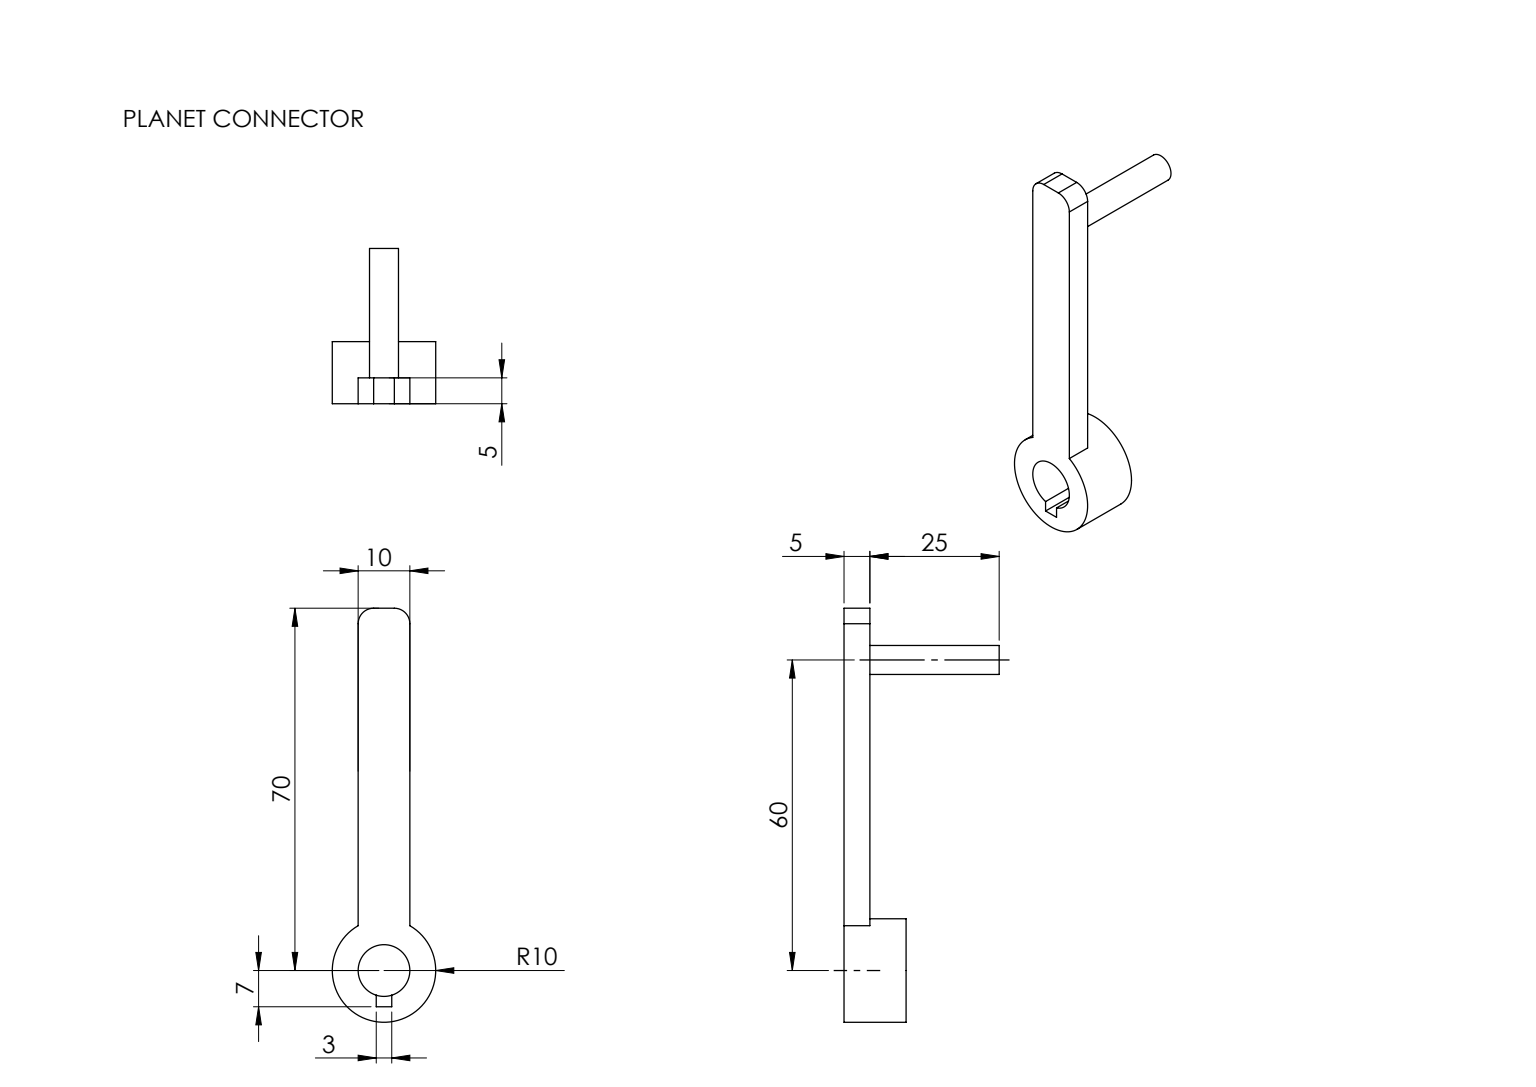
ISO-10303-21;
HEADER;
FILE_DESCRIPTION (('STEP AP214'),
    '1' );
FILE_NAME ('planet connector.step',
    '2026-09-30T13:58:28',
    ( '' ),
    ( '' ),
    'SwSTEP 2.0',
    'SolidWorks 2026',
    '' );
FILE_SCHEMA (( 'AUTOMOTIVE_DESIGN' ));
ENDSEC;

DATA;
#12=AXIS2_PLACEMENT_3D ( 'NONE', #9946, #1451, #14823 ) ;
#81=CARTESIAN_POINT ( 'NONE',  ( -1.500000000000000000, -7.000000000000000000, 15.00000000000000000 ) ) ;
#88=CARTESIAN_POINT ( 'NONE',  ( 1.500000000000000000, -4.769696007084728073, 5.000000000000004441 ) ) ;
#89=AXIS2_PLACEMENT_3D ( 'NONE', #19050, #14810, #11160 ) ;
#115=ORIENTED_EDGE ( 'NONE', *, *, #14200, .T. ) ;
#135=CARTESIAN_POINT ( 'NONE',  ( -1.500000000000000000, -7.000000000000000000, 15.00000000000000000 ) ) ;
#237=ORIENTED_EDGE ( 'NONE', *, *, #7586, .T. ) ;
#260=ORIENTED_EDGE ( 'NONE', *, *, #20533, .T. ) ;
#316=ORIENTED_EDGE ( 'NONE', *, *, #15812, .F. ) ;
#334=ADVANCED_FACE ( 'NONE', ( #9495 ), #1106, .F. ) ;
#343=CARTESIAN_POINT ( 'NONE',  ( -5.000000000000000000, 70.00000000000000000, 9.999999999999998224 ) ) ;
#350=DIRECTION ( 'NONE',  ( 0.000000000000000000, 0.000000000000000000, 1.000000000000000000 ) ) ;
#389=VERTEX_POINT ( 'NONE', #4305 ) ;
#396=MECHANICAL_DESIGN_GEOMETRIC_PRESENTATION_REPRESENTATION('',(#1101),#5694);
#476=ORIENTED_EDGE ( 'NONE', *, *, #19100, .F. ) ;
#503=CARTESIAN_POINT ( 'NONE',  ( 6.123233995736766282E-16, -5.000000000000000000, 100.0000000000000000 ) ) ;
#544=CARTESIAN_POINT ( 'NONE',  ( 0.000000000000000000, 60.00000000000000000, -15.00000000000000000 ) ) ;
#550=CARTESIAN_POINT ( 'NONE',  ( -5.000000000000000000, 67.00000000000000000, 15.00000000000000000 ) ) ;
#604=VECTOR ( 'NONE', #20554, 1000.000000000000000 ) ;
#702=EDGE_CURVE ( 'NONE', #1080, #2507, #16323, .T. ) ;
#739=VERTEX_POINT ( 'NONE', #14558 ) ;
#746=ORIENTED_EDGE ( 'NONE', *, *, #14200, .F. ) ;
#766=EDGE_LOOP ( 'NONE', ( #18980, #17981, #8903, #8482, #6986, #6402, #13820, #2183 ) ) ;
#775=CARTESIAN_POINT ( 'NONE',  ( -5.000000000000000000, 8.660254037844385522, 15.00000000000000000 ) ) ;
#779=DIRECTION ( 'NONE',  ( 1.000000000000000000, 0.000000000000000000, 0.000000000000000000 ) ) ;
#848=ORIENTED_EDGE ( 'NONE', *, *, #1999, .T. ) ;
#895=CIRCLE ( 'NONE', #21377, 3.000000000000000000 ) ;
#908=EDGE_CURVE ( 'NONE', #14453, #1080, #8374, .T. ) ;
#1010=CARTESIAN_POINT ( 'NONE',  ( 0.000000000000000000, 0.000000000000000000, 3.000000000000002665 ) ) ;
#1017=DIRECTION ( 'NONE',  ( 0.000000000000000000, 0.000000000000000000, -1.000000000000000000 ) ) ;
#1053=SURFACE_SIDE_STYLE ('',( #9425 ) ) ;
#1074=DIRECTION ( 'NONE',  ( 1.000000000000000000, 0.000000000000000000, 0.000000000000000000 ) ) ;
#1080=VERTEX_POINT ( 'NONE', #13876 ) ;
#1101=STYLED_ITEM ( 'NONE', ( #19496 ), #2505 ) ;
#1106=CYLINDRICAL_SURFACE ( 'NONE', #89, 5.000000000000000000 ) ;
#1115=DIRECTION ( 'NONE',  ( 0.000000000000000000, 0.000000000000000000, 1.000000000000000000 ) ) ;
#1188=CARTESIAN_POINT ( 'NONE',  ( 0.000000000000000000, 0.000000000000000000, 15.00000000000000000 ) ) ;
#1211=ORIENTED_EDGE ( 'NONE', *, *, #13563, .T. ) ;
#1212=EDGE_LOOP ( 'NONE', ( #11385, #19304, #21352, #17034, #4762, #16287, #21311, #7511 ) ) ;
#1224=SURFACE_STYLE_USAGE ( .BOTH. , #18251 ) ;
#1237=VECTOR ( 'NONE', #13828, 1000.000000000000000 ) ;
#1275=EDGE_CURVE ( 'NONE', #14473, #11791, #3046, .T. ) ;
#1337=DIRECTION ( 'NONE',  ( -0.000000000000000000, -0.000000000000000000, -1.000000000000000000 ) ) ;
#1380=CARTESIAN_POINT ( 'NONE',  ( 5.000000000000000000, 8.660254037844385522, 15.00000000000000000 ) ) ;
#1388=VERTEX_POINT ( 'NONE', #18623 ) ;
#1451=DIRECTION ( 'NONE',  ( 0.000000000000000000, 0.000000000000000000, -1.000000000000000000 ) ) ;
#1470=EDGE_CURVE ( 'NONE', #11833, #2563, #5467, .T. ) ;
#1473=CYLINDRICAL_SURFACE ( 'NONE', #18362, 2.799999999999996714 ) ;
#1478=ORIENTED_EDGE ( 'NONE', *, *, #2597, .T. ) ;
#1521=EDGE_CURVE ( 'NONE', #19720, #739, #10639, .T. ) ;
#1551=FACE_OUTER_BOUND ( 'NONE', #20491, .T. ) ;
#1563=ORIENTED_EDGE ( 'NONE', *, *, #13508, .T. ) ;
#1585=DIRECTION ( 'NONE',  ( 1.000000000000000000, 0.000000000000000000, 0.000000000000000000 ) ) ;
#1638=EDGE_CURVE ( 'NONE', #11791, #13591, #21809, .T. ) ;
#1665=FACE_OUTER_BOUND ( 'NONE', #12587, .T. ) ;
#1717=DIRECTION ( 'NONE',  ( -0.000000000000000000, -0.000000000000000000, -1.000000000000000000 ) ) ;
#1757=ORIENTED_EDGE ( 'NONE', *, *, #2328, .F. ) ;
#1791=PRODUCT_CONTEXT ( 'NONE', #13199, 'mechanical' ) ;
#1871=CIRCLE ( 'NONE', #14212, 2.799999999999996714 ) ;
#1876=CARTESIAN_POINT ( 'NONE',  ( 0.000000000000000000, 5.000000000000000000, 100.0000000000000000 ) ) ;
#1965=DIRECTION ( 'NONE',  ( -0.000000000000000000, 1.000000000000000000, 0.000000000000000000 ) ) ;
#1987=CARTESIAN_POINT ( 'NONE',  ( 2.000000000000000000, 67.00000000000000000, 9.999999999999998224 ) ) ;
#1999=EDGE_CURVE ( 'NONE', #2507, #2130, #17691, .T. ) ;
#2062=ORIENTED_EDGE ( 'NONE', *, *, #15004, .F. ) ;
#2119=DIRECTION ( 'NONE',  ( -0.000000000000000000, -0.000000000000000000, 1.000000000000000000 ) ) ;
#2130=VERTEX_POINT ( 'NONE', #19672 ) ;
#2133=ORIENTED_EDGE ( 'NONE', *, *, #21365, .T. ) ;
#2172=DIRECTION ( 'NONE',  ( -0.000000000000000000, -0.000000000000000000, -1.000000000000000000 ) ) ;
#2183=ORIENTED_EDGE ( 'NONE', *, *, #20898, .T. ) ;
#2197=DIRECTION ( 'NONE',  ( -0.000000000000000000, 1.000000000000000000, 0.000000000000000000 ) ) ;
#2296=ORIENTED_EDGE ( 'NONE', *, *, #8034, .T. ) ;
#2328=EDGE_CURVE ( 'NONE', #15305, #18649, #12398, .T. ) ;
#2371=CARTESIAN_POINT ( 'NONE',  ( 0.000000000000000000, 0.000000000000000000, 3.000000000000000000 ) ) ;
#2439=EDGE_CURVE ( 'NONE', #13824, #19161, #4268, .T. ) ;
#2498=FACE_OUTER_BOUND ( 'NONE', #21546, .T. ) ;
#2504=COLOUR_RGB ( '', 0.72549020, 0.75294118, 0.79215686) ;
#2505=ADVANCED_BREP_SHAPE_REPRESENTATION ( '', ( #13597, #15567 ), #16627 ) ;
#2507=VERTEX_POINT ( 'NONE', #14319 ) ;
#2555=VERTEX_POINT ( 'NONE', #11878 ) ;
#2563=VERTEX_POINT ( 'NONE', #3050 ) ;
#2597=EDGE_CURVE ( 'NONE', #4038, #20275, #16853, .T. ) ;
#2606=EDGE_CURVE ( 'NONE', #15305, #16104, #18194, .T. ) ;
#2618=DIRECTION ( 'NONE',  ( 0.000000000000000000, 0.000000000000000000, 1.000000000000000000 ) ) ;
#2657=CARTESIAN_POINT ( 'NONE',  ( 0.000000000000000000, 0.000000000000000000, 9.999999999999998224 ) ) ;
#2715=DIRECTION ( 'NONE',  ( -1.000000000000000000, 0.000000000000000000, -0.000000000000000000 ) ) ;
#2759=ORIENTED_EDGE ( 'NONE', *, *, #4928, .T. ) ;
#2808=FACE_OUTER_BOUND ( 'NONE', #17080, .T. ) ;
#2810=DIRECTION ( 'NONE',  ( -0.000000000000000000, -0.000000000000000000, 1.000000000000000000 ) ) ;
#2819=CARTESIAN_POINT ( 'NONE',  ( 0.000000000000000000, 0.000000000000000000, 3.000000000000000000 ) ) ;
#2820=ORIENTED_EDGE ( 'NONE', *, *, #17323, .T. ) ;
#2849=VERTEX_POINT ( 'NONE', #14619 ) ;
#2908=LINE ( 'NONE', #3024, #8757 ) ;
#2917=( NAMED_UNIT ( * ) SI_UNIT ( $, .STERADIAN. ) SOLID_ANGLE_UNIT ( ) );
#2953=DIRECTION ( 'NONE',  ( 1.000000000000000000, 0.000000000000000000, 0.000000000000000000 ) ) ;
#3014=DIRECTION ( 'NONE',  ( 0.000000000000000000, 0.000000000000000000, 1.000000000000000000 ) ) ;
#3024=CARTESIAN_POINT ( 'NONE',  ( 1.500000000000000000, -7.000000000000000000, 15.00000000000000000 ) ) ;
#3030=CARTESIAN_POINT ( 'NONE',  ( 0.000000000000000000, 0.000000000000000000, 15.00000000000000000 ) ) ;
#3046=LINE ( 'NONE', #15073, #18985 ) ;
#3050=CARTESIAN_POINT ( 'NONE',  ( -1.500000000000000000, -7.000000000000000000, 15.00000000000000000 ) ) ;
#3205=( LENGTH_UNIT ( ) NAMED_UNIT ( * ) SI_UNIT ( .MILLI., .METRE. ) );
#3208=VECTOR ( 'NONE', #6810, 1000.000000000000000 ) ;
#3234=EDGE_CURVE ( 'NONE', #20275, #1388, #18810, .T. ) ;
#3241=PRODUCT_DEFINITION_FORMATION_WITH_SPECIFIED_SOURCE ( 'ANY', '', #18138, .NOT_KNOWN. ) ;
#3250=CARTESIAN_POINT ( 'NONE',  ( -9.999999999999998224, 0.000000000000000000, 15.00000000000000000 ) ) ;
#3262=EDGE_CURVE ( 'NONE', #4329, #2849, #18630, .T. ) ;
#3278=ADVANCED_FACE ( 'NONE', ( #21122 ), #19130, .T. ) ;
#3281=FACE_OUTER_BOUND ( 'NONE', #20162, .T. ) ;
#3340=PRODUCT_DEFINITION ( 'UNKNOWN', '', #3241, #15569 ) ;
#3377=CYLINDRICAL_SURFACE ( 'NONE', #4800, 3.000000000000000000 ) ;
#3401=CIRCLE ( 'NONE', #6231, 5.000000000000000000 ) ;
#3539=PLANE ( 'NONE',  #9399 ) ;
#3634=EDGE_CURVE ( 'NONE', #19720, #11833, #10375, .T. ) ;
#3686=CARTESIAN_POINT ( 'NONE',  ( 0.000000000000000000, 60.00000000000000000, -15.00000000000000000 ) ) ;
#3758=CIRCLE ( 'NONE', #17537, 5.000000000000000000 ) ;
#3770=VECTOR ( 'NONE', #13636, 1000.000000000000000 ) ;
#3894=CIRCLE ( 'NONE', #12, 3.000000000000000000 ) ;
#4025=FACE_OUTER_BOUND ( 'NONE', #13212, .T. ) ;
#4027=DIRECTION ( 'NONE',  ( 1.000000000000000000, 0.000000000000000000, 0.000000000000000000 ) ) ;
#4037=ADVANCED_FACE ( 'NONE', ( #16077 ), #19617, .T. ) ;
#4038=VERTEX_POINT ( 'NONE', #14197 ) ;
#4100=ORIENTED_EDGE ( 'NONE', *, *, #1521, .F. ) ;
#4123=COLOUR_RGB ( '', 0.72549020, 0.75294118, 0.79215686) ;
#4124=CARTESIAN_POINT ( 'NONE',  ( 0.000000000000000000, 60.00000000000000000, -15.00000000000000000 ) ) ;
#4163=CARTESIAN_POINT ( 'NONE',  ( 0.000000000000000000, 0.000000000000000000, 15.00000000000000000 ) ) ;
#4268=LINE ( 'NONE', #12548, #5970 ) ;
#4281=CARTESIAN_POINT ( 'NONE',  ( 1.500000000000000000, 0.000000000000000000, 15.00000000000000000 ) ) ;
#4288=EDGE_CURVE ( 'NONE', #9061, #5771, #8054, .T. ) ;
#4302=CARTESIAN_POINT ( 'NONE',  ( -5.000000000000000000, 8.660254037844385522, 9.999999999999998224 ) ) ;
#4305=CARTESIAN_POINT ( 'NONE',  ( 1.500000000000000000, -7.000000000000000000, 15.00000000000000000 ) ) ;
#4329=VERTEX_POINT ( 'NONE', #18707 ) ;
#4377=ORIENTED_EDGE ( 'NONE', *, *, #20533, .F. ) ;
#4414=VERTEX_POINT ( 'NONE', #4302 ) ;
#4456=CARTESIAN_POINT ( 'NONE',  ( 0.000000000000000000, 0.000000000000000000, 15.00000000000000000 ) ) ;
#4482=DIRECTION ( 'NONE',  ( -0.000000000000000000, -0.000000000000000000, -1.000000000000000000 ) ) ;
#4551=CARTESIAN_POINT ( 'NONE',  ( 2.000000000000000000, 67.00000000000000000, 9.999999999999998224 ) ) ;
#4624=DIRECTION ( 'NONE',  ( 0.000000000000000000, 0.000000000000000000, 1.000000000000000000 ) ) ;
#4669=PLANE ( 'NONE',  #21706 ) ;
#4725=DIRECTION ( 'NONE',  ( 0.000000000000000000, 0.000000000000000000, 1.000000000000000000 ) ) ;
#4743=AXIS2_PLACEMENT_3D ( 'NONE', #3686, #16628, #13304 ) ;
#4757=FILL_AREA_STYLE ('',( #8185 ) ) ;
#4762=ORIENTED_EDGE ( 'NONE', *, *, #7302, .F. ) ;
#4800=AXIS2_PLACEMENT_3D ( 'NONE', #8567, #11993, #20899 ) ;
#4805=ORIENTED_EDGE ( 'NONE', *, *, #2439, .F. ) ;
#4860=AXIS2_PLACEMENT_3D ( 'NONE', #12427, #4482, #21170 ) ;
#4872=DIRECTION ( 'NONE',  ( -0.000000000000000000, -0.000000000000000000, 1.000000000000000000 ) ) ;
#4880=VECTOR ( 'NONE', #15733, 1000.000000000000000 ) ;
#4902=DIRECTION ( 'NONE',  ( 0.000000000000000000, 0.000000000000000000, -1.000000000000000000 ) ) ;
#4928=EDGE_CURVE ( 'NONE', #14192, #2555, #15485, .T. ) ;
#4949=EDGE_LOOP ( 'NONE', ( #7138, #316, #5329, #16978, #14225 ) ) ;
#5034=ADVANCED_FACE ( 'NONE', ( #6733 ), #13335, .T. ) ;
#5053=DIRECTION ( 'NONE',  ( -0.000000000000000000, 0.000000000000000000, -1.000000000000000000 ) ) ;
#5055=CARTESIAN_POINT ( 'NONE',  ( -1.500000000000000000, 0.000000000000000000, 15.00000000000000000 ) ) ;
#5192=( GEOMETRIC_REPRESENTATION_CONTEXT ( 3 ) GLOBAL_UNCERTAINTY_ASSIGNED_CONTEXT ( ( #7912 ) ) GLOBAL_UNIT_ASSIGNED_CONTEXT ( ( #3205, #18687, #16799 ) ) REPRESENTATION_CONTEXT ( 'NONE', 'WORKASPACE' ) );
#5261=CARTESIAN_POINT ( 'NONE',  ( 0.000000000000000000, 0.000000000000000000, 15.00000000000000000 ) ) ;
#5329=ORIENTED_EDGE ( 'NONE', *, *, #4928, .F. ) ;
#5369=DIRECTION ( 'NONE',  ( 0.000000000000000000, 0.000000000000000000, -1.000000000000000000 ) ) ;
#5415=DIRECTION ( 'NONE',  ( -0.000000000000000000, 0.000000000000000000, -1.000000000000000000 ) ) ;
#5467=LINE ( 'NONE', #7021, #3770 ) ;
#5485=AXIS2_PLACEMENT_3D ( 'NONE', #135, #8532, #10292 ) ;
#5543=VECTOR ( 'NONE', #7083, 1000.000000000000000 ) ;
#5694=( GEOMETRIC_REPRESENTATION_CONTEXT ( 3 ) GLOBAL_UNCERTAINTY_ASSIGNED_CONTEXT ( ( #13198 ) ) GLOBAL_UNIT_ASSIGNED_CONTEXT ( ( #14525, #12971, #2917 ) ) REPRESENTATION_CONTEXT ( 'NONE', 'WORKASPACE' ) );
#5771=VERTEX_POINT ( 'NONE', #12923 ) ;
#5842=ORIENTED_EDGE ( 'NONE', *, *, #19542, .F. ) ;
#5913=EDGE_LOOP ( 'NONE', ( #12862, #1563, #21194, #746 ) ) ;
#5953=ADVANCED_FACE ( 'NONE', ( #15568 ), #10482, .T. ) ;
#5970=VECTOR ( 'NONE', #6156, 1000.000000000000000 ) ;
#5992=DIRECTION ( 'NONE',  ( -0.000000000000000000, -0.000000000000000000, -1.000000000000000000 ) ) ;
#5997=EDGE_CURVE ( 'NONE', #7490, #19853, #15622, .T. ) ;
#6028=CIRCLE ( 'NONE', #12706, 3.000000000000000000 ) ;
#6049=VECTOR ( 'NONE', #18416, 1000.000000000000000 ) ;
#6156=DIRECTION ( 'NONE',  ( -0.000000000000000000, -0.000000000000000000, -1.000000000000000000 ) ) ;
#6231=AXIS2_PLACEMENT_3D ( 'NONE', #13918, #350, #9050 ) ;
#6238=FACE_OUTER_BOUND ( 'NONE', #1212, .T. ) ;
#6251=MECHANICAL_DESIGN_GEOMETRIC_PRESENTATION_REPRESENTATION('',(#15762),#5192);
#6256=ORIENTED_EDGE ( 'NONE', *, *, #21132, .F. ) ;
#6350=AXIS2_PLACEMENT_3D ( 'NONE', #4163, #7151, #20630 ) ;
#6402=ORIENTED_EDGE ( 'NONE', *, *, #10568, .F. ) ;
#6413=CARTESIAN_POINT ( 'NONE',  ( 0.000000000000000000, 60.00000000000000000, 9.999999999999998224 ) ) ;
#6484=CARTESIAN_POINT ( 'NONE',  ( 1.500000000000000000, 0.000000000000000000, 5.000000000000000000 ) ) ;
#6541=DIRECTION ( 'NONE',  ( 0.000000000000000000, -1.000000000000000000, 0.000000000000000000 ) ) ;
#6578=DIRECTION ( 'NONE',  ( 1.000000000000000000, 0.000000000000000000, 0.000000000000000000 ) ) ;
#6597=CARTESIAN_POINT ( 'NONE',  ( 5.000000000000000000, 5.000000000000000000, 9.999999999999998224 ) ) ;
#6626=CARTESIAN_POINT ( 'NONE',  ( -9.999999999999998224, 0.000000000000000000, 15.00000000000000000 ) ) ;
#6655=PLANE ( 'NONE',  #9820 ) ;
#6694=DIRECTION ( 'NONE',  ( -0.000000000000000000, -0.000000000000000000, 1.000000000000000000 ) ) ;
#6733=FACE_OUTER_BOUND ( 'NONE', #11550, .T. ) ;
#6779=PLANE ( 'NONE',  #5485 ) ;
#6787=VECTOR ( 'NONE', #4725, 1000.000000000000000 ) ;
#6810=DIRECTION ( 'NONE',  ( -0.000000000000000000, 1.000000000000000000, 0.000000000000000000 ) ) ;
#6954=CARTESIAN_POINT ( 'NONE',  ( 5.000000000000000000, 5.000000000000000000, 15.00000000000000000 ) ) ;
#6986=ORIENTED_EDGE ( 'NONE', *, *, #16829, .F. ) ;
#7021=CARTESIAN_POINT ( 'NONE',  ( -1.500000000000000000, 0.000000000000000000, 15.00000000000000000 ) ) ;
#7027=ORIENTED_EDGE ( 'NONE', *, *, #16988, .T. ) ;
#7047=ORIENTED_EDGE ( 'NONE', *, *, #2606, .F. ) ;
#7083=DIRECTION ( 'NONE',  ( 1.000000000000000000, 0.000000000000000000, 0.000000000000000000 ) ) ;
#7115=ORIENTED_EDGE ( 'NONE', *, *, #13249, .T. ) ;
#7138=ORIENTED_EDGE ( 'NONE', *, *, #1470, .F. ) ;
#7151=DIRECTION ( 'NONE',  ( -0.000000000000000000, -0.000000000000000000, -1.000000000000000000 ) ) ;
#7166=ORIENTED_EDGE ( 'NONE', *, *, #3634, .F. ) ;
#7211=DIRECTION ( 'NONE',  ( 0.000000000000000000, 0.000000000000000000, 1.000000000000000000 ) ) ;
#7266=AXIS2_PLACEMENT_3D ( 'NONE', #5261, #18522, #12493 ) ;
#7292=ADVANCED_FACE ( 'NONE', ( #14021 ), #20553, .F. ) ;
#7302=EDGE_CURVE ( 'NONE', #21336, #13824, #10600, .T. ) ;
#7320=LINE ( 'NONE', #775, #1237 ) ;
#7400=DIRECTION ( 'NONE',  ( -1.000000000000000000, 0.000000000000000000, 0.000000000000000000 ) ) ;
#7435=CARTESIAN_POINT ( 'NONE',  ( 6.123233995736766282E-16, -5.000000000000000000, 5.000000000000004441 ) ) ;
#7465=ORIENTED_EDGE ( 'NONE', *, *, #20383, .F. ) ;
#7490=VERTEX_POINT ( 'NONE', #16447 ) ;
#7491=ORIENTED_EDGE ( 'NONE', *, *, #7549, .T. ) ;
#7511=ORIENTED_EDGE ( 'NONE', *, *, #20997, .T. ) ;
#7537=EDGE_LOOP ( 'NONE', ( #18748, #21165 ) ) ;
#7549=EDGE_CURVE ( 'NONE', #5771, #9061, #15617, .T. ) ;
#7586=EDGE_CURVE ( 'NONE', #8720, #13591, #18340, .T. ) ;
#7605=EDGE_CURVE ( 'NONE', #8443, #1388, #21855, .T. ) ;
#7710=CARTESIAN_POINT ( 'NONE',  ( -2.000000000000000000, 67.00000000000000000, 15.00000000000000000 ) ) ;
#7738=VECTOR ( 'NONE', #8615, 1000.000000000000000 ) ;
#7739=ORIENTED_EDGE ( 'NONE', *, *, #4288, .T. ) ;
#7757=DIRECTION ( 'NONE',  ( 1.000000000000000000, 0.000000000000000000, 0.000000000000000000 ) ) ;
#7782=CARTESIAN_POINT ( 'NONE',  ( 0.000000000000000000, 0.000000000000000000, 100.0000000000000000 ) ) ;
#7855=AXIS2_PLACEMENT_3D ( 'NONE', #544, #20766, #20650 ) ;
#7912=UNCERTAINTY_MEASURE_WITH_UNIT (LENGTH_MEASURE( 1.000000000000000082E-05 ), #3205, 'distance_accuracy_value', 'NONE');
#7924=EDGE_LOOP ( 'NONE', ( #8411, #7465, #12128, #12619 ) ) ;
#8007=EDGE_CURVE ( 'NONE', #19853, #7490, #1871, .T. ) ;
#8034=EDGE_CURVE ( 'NONE', #15305, #14192, #17609, .T. ) ;
#8054=CIRCLE ( 'NONE', #9799, 2.799999999999996714 ) ;
#8148=CARTESIAN_POINT ( 'NONE',  ( -5.000000000000000000, 5.000000000000000000, 9.999999999999998224 ) ) ;
#8185=FILL_AREA_STYLE_COLOUR ( '', #4123 ) ;
#8215=CARTESIAN_POINT ( 'NONE',  ( 0.000000000000000000, 60.00000000000000000, -15.00000000000000000 ) ) ;
#8282=ADVANCED_FACE ( 'NONE', ( #3281 ), #10012, .F. ) ;
#8284=ORIENTED_EDGE ( 'NONE', *, *, #908, .F. ) ;
#8298=CARTESIAN_POINT ( 'NONE',  ( 0.000000000000000000, 0.000000000000000000, 5.000000000000000000 ) ) ;
#8368=DIRECTION ( 'NONE',  ( 1.000000000000000000, 0.000000000000000000, -0.000000000000000000 ) ) ;
#8372=DIRECTION ( 'NONE',  ( 0.000000000000000000, 1.000000000000000000, 0.000000000000000000 ) ) ;
#8374=LINE ( 'NONE', #9913, #6787 ) ;
#8408=CARTESIAN_POINT ( 'NONE',  ( 5.000000000000000000, 5.000000000000000000, 9.999999999999998224 ) ) ;
#8411=ORIENTED_EDGE ( 'NONE', *, *, #13249, .F. ) ;
#8440=LINE ( 'NONE', #20252, #13538 ) ;
#8443=VERTEX_POINT ( 'NONE', #11216 ) ;
#8482=ORIENTED_EDGE ( 'NONE', *, *, #7586, .F. ) ;
#8532=DIRECTION ( 'NONE',  ( 0.000000000000000000, 1.000000000000000000, 0.000000000000000000 ) ) ;
#8535=CARTESIAN_POINT ( 'NONE',  ( -1.500000000000000000, -7.000000000000000000, 5.000000000000000000 ) ) ;
#8547=ORIENTED_EDGE ( 'NONE', *, *, #7302, .T. ) ;
#8567=CARTESIAN_POINT ( 'NONE',  ( -2.000000000000000000, 67.00000000000000000, 9.999999999999998224 ) ) ;
#8615=DIRECTION ( 'NONE',  ( 0.000000000000000000, 0.000000000000000000, -1.000000000000000000 ) ) ;
#8625=AXIS2_PLACEMENT_3D ( 'NONE', #10374, #20870, #12144 ) ;
#8690=ORIENTED_EDGE ( 'NONE', *, *, #20898, .F. ) ;
#8709=ADVANCED_FACE ( 'NONE', ( #18831 ), #18505, .T. ) ;
#8720=VERTEX_POINT ( 'NONE', #3250 ) ;
#8723=EDGE_LOOP ( 'NONE', ( #17316, #18211, #6256, #16096 ) ) ;
#8730=LINE ( 'NONE', #343, #5543 ) ;
#8757=VECTOR ( 'NONE', #18278, 1000.000000000000000 ) ;
#8903=ORIENTED_EDGE ( 'NONE', *, *, #1638, .T. ) ;
#8908=VECTOR ( 'NONE', #13342, 1000.000000000000000 ) ;
#9013=CIRCLE ( 'NONE', #7266, 9.999999999999998224 ) ;
#9017=CYLINDRICAL_SURFACE ( 'NONE', #6350, 9.999999999999998224 ) ;
#9023=CARTESIAN_POINT ( 'NONE',  ( -1.500000000000000000, -7.000000000000000000, 15.00000000000000000 ) ) ;
#9050=DIRECTION ( 'NONE',  ( 1.000000000000000000, 0.000000000000000000, 0.000000000000000000 ) ) ;
#9061=VERTEX_POINT ( 'NONE', #15049 ) ;
#9069=CARTESIAN_POINT ( 'NONE',  ( -1.500000000000000000, -4.769696007084728073, 15.00000000000000000 ) ) ;
#9116=ORIENTED_EDGE ( 'NONE', *, *, #3262, .F. ) ;
#9118=ORIENTED_EDGE ( 'NONE', *, *, #2597, .F. ) ;
#9224=CARTESIAN_POINT ( 'NONE',  ( 0.000000000000000000, 0.000000000000000000, 9.999999999999998224 ) ) ;
#9234=DIRECTION ( 'NONE',  ( 0.000000000000000000, 0.000000000000000000, -1.000000000000000000 ) ) ;
#9319=( NAMED_UNIT ( * ) SI_UNIT ( $, .STERADIAN. ) SOLID_ANGLE_UNIT ( ) );
#9399=AXIS2_PLACEMENT_3D ( 'NONE', #8408, #20552, #5415 ) ;
#9417=ORIENTED_EDGE ( 'NONE', *, *, #2439, .T. ) ;
#9425=SURFACE_STYLE_FILL_AREA ( #12751 ) ;
#9433=EDGE_CURVE ( 'NONE', #8720, #14473, #18881, .T. ) ;
#9455=LINE ( 'NONE', #8148, #15490 ) ;
#9495=FACE_OUTER_BOUND ( 'NONE', #17817, .T. ) ;
#9555=ORIENTED_EDGE ( 'NONE', *, *, #21365, .F. ) ;
#9578=EDGE_CURVE ( 'NONE', #2563, #389, #12010, .T. ) ;
#9632=CYLINDRICAL_SURFACE ( 'NONE', #11420, 5.000000000000000000 ) ;
#9761=( LENGTH_UNIT ( ) NAMED_UNIT ( * ) SI_UNIT ( .MILLI., .METRE. ) );
#9794=DIRECTION ( 'NONE',  ( 0.000000000000000000, 0.000000000000000000, 1.000000000000000000 ) ) ;
#9799=AXIS2_PLACEMENT_3D ( 'NONE', #17258, #2119, #12055 ) ;
#9820=AXIS2_PLACEMENT_3D ( 'NONE', #8298, #1115, #16355 ) ;
#9829=PRESENTATION_STYLE_ASSIGNMENT (( #1224 ) ) ;
#9834=CIRCLE ( 'NONE', #19370, 3.000000000000000000 ) ;
#9913=CARTESIAN_POINT ( 'NONE',  ( -2.000000000000000000, 70.00000000000000000, 9.999999999999998224 ) ) ;
#9946=CARTESIAN_POINT ( 'NONE',  ( -2.000000000000000000, 67.00000000000000000, 9.999999999999998224 ) ) ;
#9967=VECTOR ( 'NONE', #1965, 1000.000000000000000 ) ;
#10012=PLANE ( 'NONE',  #18485 ) ;
#10046=AXIS2_PLACEMENT_3D ( 'NONE', #4281, #11016, #17769 ) ;
#10109=AXIS2_PLACEMENT_3D ( 'NONE', #2657, #12711, #12278 ) ;
#10203=AXIS2_PLACEMENT_3D ( 'NONE', #2819, #11207, #4027 ) ;
#10273=ADVANCED_FACE ( 'NONE', ( #6238, #19476 ), #4669, .T. ) ;
#10275=LINE ( 'NONE', #1876, #7738 ) ;
#10292=DIRECTION ( 'NONE',  ( -1.000000000000000000, 0.000000000000000000, 0.000000000000000000 ) ) ;
#10374=CARTESIAN_POINT ( 'NONE',  ( -5.000000000000000000, 70.00000000000000000, 9.999999999999998224 ) ) ;
#10375=LINE ( 'NONE', #10490, #604 ) ;
#10397=FACE_OUTER_BOUND ( 'NONE', #7924, .T. ) ;
#10442=ADVANCED_FACE ( 'NONE', ( #10397 ), #6779, .T. ) ;
#10478=EDGE_LOOP ( 'NONE', ( #16127, #848, #15097, #18321 ) ) ;
#10482=CYLINDRICAL_SURFACE ( 'NONE', #12793, 3.000000000000000000 ) ;
#10488=CARTESIAN_POINT ( 'NONE',  ( -5.000000000000000000, 5.000000000000000000, 15.00000000000000000 ) ) ;
#10490=CARTESIAN_POINT ( 'NONE',  ( -1.500000000000000000, -4.769696007084728073, 100.0000000000000000 ) ) ;
#10506=ORIENTED_EDGE ( 'NONE', *, *, #10568, .T. ) ;
#10511=CARTESIAN_POINT ( 'NONE',  ( 9.999999999999998224, 1.224646799147353059E-15, 3.000000000000000000 ) ) ;
#10568=EDGE_CURVE ( 'NONE', #4414, #21336, #7320, .T. ) ;
#10600=LINE ( 'NONE', #10488, #19565 ) ;
#10639=LINE ( 'NONE', #17392, #4880 ) ;
#10897=VECTOR ( 'NONE', #9234, 1000.000000000000000 ) ;
#11001=FACE_BOUND ( 'NONE', #16075, .T. ) ;
#11016=DIRECTION ( 'NONE',  ( 1.000000000000000000, 0.000000000000000000, 0.000000000000000000 ) ) ;
#11134=EDGE_LOOP ( 'NONE', ( #12698, #11630, #17145, #17359 ) ) ;
#11160=DIRECTION ( 'NONE',  ( 0.000000000000000000, 1.000000000000000000, 0.000000000000000000 ) ) ;
#11207=DIRECTION ( 'NONE',  ( 0.000000000000000000, 0.000000000000000000, 1.000000000000000000 ) ) ;
#11216=CARTESIAN_POINT ( 'NONE',  ( 5.000000000000000000, 8.660254037844385522, 15.00000000000000000 ) ) ;
#11281=AXIS2_PLACEMENT_3D ( 'NONE', #3030, #21804, #1585 ) ;
#11329=ORIENTED_EDGE ( 'NONE', *, *, #13691, .T. ) ;
#11349=CARTESIAN_POINT ( 'NONE',  ( -5.000000000000000000, 70.00000000000000000, 15.00000000000000000 ) ) ;
#11385=ORIENTED_EDGE ( 'NONE', *, *, #7605, .T. ) ;
#11420=AXIS2_PLACEMENT_3D ( 'NONE', #7782, #4902, #13287 ) ;
#11542=ADVANCED_FACE ( 'NONE', ( #2808 ), #9632, .F. ) ;
#11550=EDGE_LOOP ( 'NONE', ( #21315, #14593, #16042, #4100 ) ) ;
#11581=DIRECTION ( 'NONE',  ( 1.000000000000000000, 0.000000000000000000, 0.000000000000000000 ) ) ;
#11630=ORIENTED_EDGE ( 'NONE', *, *, #14325, .F. ) ;
#11677=EDGE_CURVE ( 'NONE', #14192, #389, #8440, .T. ) ;
#11750=CARTESIAN_POINT ( 'NONE',  ( -1.500000000000000000, -4.769696007084728073, 5.000000000000004441 ) ) ;
#11791=VERTEX_POINT ( 'NONE', #10511 ) ;
#11833=VERTEX_POINT ( 'NONE', #9069 ) ;
#11878=CARTESIAN_POINT ( 'NONE',  ( 0.000000000000000000, 5.000000000000000000, 15.00000000000000000 ) ) ;
#11971=FACE_OUTER_BOUND ( 'NONE', #5913, .T. ) ;
#11993=DIRECTION ( 'NONE',  ( 0.000000000000000000, 0.000000000000000000, 1.000000000000000000 ) ) ;
#12004=ORIENTED_EDGE ( 'NONE', *, *, #17323, .F. ) ;
#12010=LINE ( 'NONE', #81, #14253 ) ;
#12055=DIRECTION ( 'NONE',  ( -1.000000000000000000, 0.000000000000000000, 0.000000000000000000 ) ) ;
#12057=ADVANCED_FACE ( 'NONE', ( #21084 ), #19419, .F. ) ;
#12100=ORIENTED_EDGE ( 'NONE', *, *, #2328, .T. ) ;
#12128=ORIENTED_EDGE ( 'NONE', *, *, #9578, .T. ) ;
#12144=DIRECTION ( 'NONE',  ( 0.000000000000000000, -0.000000000000000000, -1.000000000000000000 ) ) ;
#12190=DIRECTION ( 'NONE',  ( -1.000000000000000000, 0.000000000000000000, 0.000000000000000000 ) ) ;
#12214=DIRECTION ( 'NONE',  ( 0.000000000000000000, 0.000000000000000000, 1.000000000000000000 ) ) ;
#12237=LINE ( 'NONE', #9023, #10897 ) ;
#12278=DIRECTION ( 'NONE',  ( -1.000000000000000000, 0.000000000000000000, 0.000000000000000000 ) ) ;
#12386=DIRECTION ( 'NONE',  ( 0.000000000000000000, 0.000000000000000000, 1.000000000000000000 ) ) ;
#12398=CIRCLE ( 'NONE', #15225, 5.000000000000000000 ) ;
#12427=CARTESIAN_POINT ( 'NONE',  ( 0.000000000000000000, 0.000000000000000000, 15.00000000000000000 ) ) ;
#12493=DIRECTION ( 'NONE',  ( 1.000000000000000000, 0.000000000000000000, 0.000000000000000000 ) ) ;
#12512=DIRECTION ( 'NONE',  ( 0.000000000000000000, 0.000000000000000000, 1.000000000000000000 ) ) ;
#12548=CARTESIAN_POINT ( 'NONE',  ( -5.000000000000000000, 67.00000000000000000, 9.999999999999998224 ) ) ;
#12576=ADVANCED_FACE ( 'NONE', ( #11001, #2498 ), #16082, .T. ) ;
#12587=EDGE_LOOP ( 'NONE', ( #1478, #18564, #15099, #8690 ) ) ;
#12619=ORIENTED_EDGE ( 'NONE', *, *, #14325, .T. ) ;
#12698=ORIENTED_EDGE ( 'NONE', *, *, #2606, .T. ) ;
#12706=AXIS2_PLACEMENT_3D ( 'NONE', #19138, #15500, #17497 ) ;
#12711=DIRECTION ( 'NONE',  ( 0.000000000000000000, 0.000000000000000000, -1.000000000000000000 ) ) ;
#12751=FILL_AREA_STYLE ('',( #14419 ) ) ;
#12793=AXIS2_PLACEMENT_3D ( 'NONE', #1987, #20867, #7400 ) ;
#12810=LINE ( 'NONE', #19558, #13280 ) ;
#12861=( NAMED_UNIT ( * ) PLANE_ANGLE_UNIT ( ) SI_UNIT ( $, .RADIAN. ) );
#12862=ORIENTED_EDGE ( 'NONE', *, *, #8007, .F. ) ;
#12923=CARTESIAN_POINT ( 'NONE',  ( -2.799999999999996714, 60.00000000000000000, 9.999999999999998224 ) ) ;
#12926=CARTESIAN_POINT ( 'NONE',  ( 0.000000000000000000, 0.000000000000000000, 5.000000000000004441 ) ) ;
#12971=( NAMED_UNIT ( * ) PLANE_ANGLE_UNIT ( ) SI_UNIT ( $, .RADIAN. ) );
#13089=ORIENTED_EDGE ( 'NONE', *, *, #1521, .T. ) ;
#13144=SURFACE_STYLE_FILL_AREA ( #4757 ) ;
#13152=ORIENTED_EDGE ( 'NONE', *, *, #13508, .F. ) ;
#13172=CARTESIAN_POINT ( 'NONE',  ( -2.000000000000000000, 70.00000000000000000, 9.999999999999998224 ) ) ;
#13190=EDGE_LOOP ( 'NONE', ( #9555, #4805, #476, #8284 ) ) ;
#13198=UNCERTAINTY_MEASURE_WITH_UNIT (LENGTH_MEASURE( 1.000000000000000082E-05 ), #14525, 'distance_accuracy_value', 'NONE');
#13199=APPLICATION_CONTEXT ( 'automotive_design' ) ;
#13212=EDGE_LOOP ( 'NONE', ( #5842, #13488 ) ) ;
#13249=EDGE_CURVE ( 'NONE', #739, #16104, #15594, .T. ) ;
#13280=VECTOR ( 'NONE', #4872, 1000.000000000000000 ) ;
#13287=DIRECTION ( 'NONE',  ( 0.000000000000000000, 1.000000000000000000, 0.000000000000000000 ) ) ;
#13304=DIRECTION ( 'NONE',  ( -1.000000000000000000, 0.000000000000000000, -0.000000000000000000 ) ) ;
#13316=ORIENTED_EDGE ( 'NONE', *, *, #15004, .T. ) ;
#13335=PLANE ( 'NONE',  #16918 ) ;
#13342=DIRECTION ( 'NONE',  ( -0.000000000000000000, -0.000000000000000000, -1.000000000000000000 ) ) ;
#13353=AXIS2_PLACEMENT_3D ( 'NONE', #1188, #9794, #2953 ) ;
#13387=SHAPE_DEFINITION_REPRESENTATION ( #15319, #14169 ) ;
#13392=EDGE_CURVE ( 'NONE', #4414, #4038, #17887, .T. ) ;
#13409=DIRECTION ( 'NONE',  ( 0.000000000000000000, 0.000000000000000000, 1.000000000000000000 ) ) ;
#13488=ORIENTED_EDGE ( 'NONE', *, *, #1638, .F. ) ;
#13508=EDGE_CURVE ( 'NONE', #19853, #5771, #12810, .T. ) ;
#13538=VECTOR ( 'NONE', #15493, 1000.000000000000000 ) ;
#13563=EDGE_CURVE ( 'NONE', #18649, #19720, #3758, .T. ) ;
#13575=ORIENTED_EDGE ( 'NONE', *, *, #13392, .F. ) ;
#13591=VERTEX_POINT ( 'NONE', #20010 ) ;
#13597=MANIFOLD_SOLID_BREP ( 'Fillet1', #20659 ) ;
#13636=DIRECTION ( 'NONE',  ( 0.000000000000000000, -1.000000000000000000, 0.000000000000000000 ) ) ;
#13638=ADVANCED_FACE ( 'NONE', ( #1665 ), #3539, .T. ) ;
#13691=EDGE_CURVE ( 'NONE', #14453, #2130, #8730, .T. ) ;
#13696=ORIENTED_EDGE ( 'NONE', *, *, #5997, .F. ) ;
#13741=CARTESIAN_POINT ( 'NONE',  ( -2.799999999999996714, 60.00000000000000000, -15.00000000000000000 ) ) ;
#13761=CARTESIAN_POINT ( 'NONE',  ( 0.000000000000000000, 0.000000000000000000, 15.00000000000000000 ) ) ;
#13820=ORIENTED_EDGE ( 'NONE', *, *, #13392, .T. ) ;
#13824=VERTEX_POINT ( 'NONE', #550 ) ;
#13828=DIRECTION ( 'NONE',  ( 0.000000000000000000, 0.000000000000000000, 1.000000000000000000 ) ) ;
#13833=CARTESIAN_POINT ( 'NONE',  ( 5.000000000000000000, 67.00000000000000000, 15.00000000000000000 ) ) ;
#13834=CARTESIAN_POINT ( 'NONE',  ( 9.999999999999998224, 1.224646799147353059E-15, 15.00000000000000000 ) ) ;
#13876=CARTESIAN_POINT ( 'NONE',  ( -2.000000000000000000, 70.00000000000000000, 15.00000000000000000 ) ) ;
#13918=CARTESIAN_POINT ( 'NONE',  ( 0.000000000000000000, 0.000000000000000000, 3.000000000000002665 ) ) ;
#14021=FACE_OUTER_BOUND ( 'NONE', #10478, .T. ) ;
#14169=SHAPE_REPRESENTATION ( 'planet connector', ( #15567 ), #16627 ) ;
#14192=VERTEX_POINT ( 'NONE', #16175 ) ;
#14197=CARTESIAN_POINT ( 'NONE',  ( 5.000000000000000000, 8.660254037844385522, 9.999999999999998224 ) ) ;
#14200=EDGE_CURVE ( 'NONE', #7490, #9061, #17625, .T. ) ;
#14212=AXIS2_PLACEMENT_3D ( 'NONE', #4124, #20489, #12190 ) ;
#14225=ORIENTED_EDGE ( 'NONE', *, *, #9578, .F. ) ;
#14253=VECTOR ( 'NONE', #15431, 1000.000000000000000 ) ;
#14319=CARTESIAN_POINT ( 'NONE',  ( 2.000000000000000000, 70.00000000000000000, 15.00000000000000000 ) ) ;
#14323=VECTOR ( 'NONE', #20685, 1000.000000000000000 ) ;
#14325=EDGE_CURVE ( 'NONE', #389, #16104, #2908, .T. ) ;
#14333=CARTESIAN_POINT ( 'NONE',  ( -5.000000000000000000, 67.00000000000000000, 9.999999999999998224 ) ) ;
#14391=CARTESIAN_POINT ( 'NONE',  ( 1.500000000000000000, -4.769696007084728073, 100.0000000000000000 ) ) ;
#14419=FILL_AREA_STYLE_COLOUR ( '', #2504 ) ;
#14453=VERTEX_POINT ( 'NONE', #13172 ) ;
#14473=VERTEX_POINT ( 'NONE', #13834 ) ;
#14525=( LENGTH_UNIT ( ) NAMED_UNIT ( * ) SI_UNIT ( .MILLI., .METRE. ) );
#14558=CARTESIAN_POINT ( 'NONE',  ( -1.500000000000000000, -7.000000000000000000, 5.000000000000000000 ) ) ;
#14593=ORIENTED_EDGE ( 'NONE', *, *, #1470, .T. ) ;
#14619=CARTESIAN_POINT ( 'NONE',  ( 0.000000000000000000, 5.000000000000000000, 3.000000000000002665 ) ) ;
#14756=ADVANCED_FACE ( 'NONE', ( #1551 ), #6655, .T. ) ;
#14810=DIRECTION ( 'NONE',  ( 0.000000000000000000, 0.000000000000000000, -1.000000000000000000 ) ) ;
#14815=VECTOR ( 'NONE', #13409, 1000.000000000000000 ) ;
#14823=DIRECTION ( 'NONE',  ( -1.000000000000000000, 0.000000000000000000, 0.000000000000000000 ) ) ;
#15004=EDGE_CURVE ( 'NONE', #2555, #2849, #10275, .T. ) ;
#15009=ORIENTED_EDGE ( 'NONE', *, *, #19359, .T. ) ;
#15049=CARTESIAN_POINT ( 'NONE',  ( 2.799999999999996714, 60.00000000000000000, 9.999999999999998224 ) ) ;
#15073=CARTESIAN_POINT ( 'NONE',  ( 9.999999999999998224, 1.224646799147353059E-15, 15.00000000000000000 ) ) ;
#15097=ORIENTED_EDGE ( 'NONE', *, *, #13691, .F. ) ;
#15099=ORIENTED_EDGE ( 'NONE', *, *, #7605, .F. ) ;
#15125=EDGE_LOOP ( 'NONE', ( #13152, #13696, #115, #20488 ) ) ;
#15139=AXIS2_PLACEMENT_3D ( 'NONE', #2371, #12214, #17635 ) ;
#15225=AXIS2_PLACEMENT_3D ( 'NONE', #15880, #2172, #15645 ) ;
#15305=VERTEX_POINT ( 'NONE', #88 ) ;
#15319=PRODUCT_DEFINITION_SHAPE ( 'NONE', 'NONE',  #3340 ) ;
#15329=ORIENTED_EDGE ( 'NONE', *, *, #3262, .T. ) ;
#15330=CARTESIAN_POINT ( 'NONE',  ( 5.000000000000000000, 67.00000000000000000, 9.999999999999998224 ) ) ;
#15431=DIRECTION ( 'NONE',  ( 1.000000000000000000, 0.000000000000000000, 0.000000000000000000 ) ) ;
#15485=CIRCLE ( 'NONE', #13353, 5.000000000000000000 ) ;
#15490=VECTOR ( 'NONE', #16210, 1000.000000000000000 ) ;
#15493=DIRECTION ( 'NONE',  ( 0.000000000000000000, -1.000000000000000000, 0.000000000000000000 ) ) ;
#15500=DIRECTION ( 'NONE',  ( 0.000000000000000000, 0.000000000000000000, 1.000000000000000000 ) ) ;
#15525=ADVANCED_FACE ( 'NONE', ( #20956 ), #9017, .T. ) ;
#15567=AXIS2_PLACEMENT_3D ( 'NONE', #21837, #20187, #17085 ) ;
#15568=FACE_OUTER_BOUND ( 'NONE', #8723, .T. ) ;
#15569=PRODUCT_DEFINITION_CONTEXT ( 'detailed design', #17729, 'design' ) ;
#15594=LINE ( 'NONE', #8535, #14323 ) ;
#15617=CIRCLE ( 'NONE', #17746, 2.799999999999996714 ) ;
#15622=CIRCLE ( 'NONE', #7855, 2.799999999999996714 ) ;
#15645=DIRECTION ( 'NONE',  ( -3.552713678800500929E-15, -1.000000000000000000, 0.000000000000000000 ) ) ;
#15733=DIRECTION ( 'NONE',  ( 0.000000000000000000, -1.000000000000000000, 0.000000000000000000 ) ) ;
#15762=STYLED_ITEM ( 'NONE', ( #9829 ), #13597 ) ;
#15812=EDGE_CURVE ( 'NONE', #2555, #11833, #17648, .T. ) ;
#15848=CARTESIAN_POINT ( 'NONE',  ( 0.000000000000000000, 0.000000000000000000, 3.000000000000000000 ) ) ;
#15880=CARTESIAN_POINT ( 'NONE',  ( 0.000000000000000000, 0.000000000000000000, 5.000000000000004441 ) ) ;
#15896=DIRECTION ( 'NONE',  ( 1.000000000000000000, 0.000000000000000000, 0.000000000000000000 ) ) ;
#15942=DIRECTION ( 'NONE',  ( 1.000000000000000000, 0.000000000000000000, 0.000000000000000000 ) ) ;
#15978=VECTOR ( 'NONE', #18045, 1000.000000000000000 ) ;
#16042=ORIENTED_EDGE ( 'NONE', *, *, #20383, .T. ) ;
#16075=EDGE_LOOP ( 'NONE', ( #7739, #7491 ) ) ;
#16077=FACE_OUTER_BOUND ( 'NONE', #766, .T. ) ;
#16082=PLANE ( 'NONE',  #16772 ) ;
#16096=ORIENTED_EDGE ( 'NONE', *, *, #3234, .F. ) ;
#16104=VERTEX_POINT ( 'NONE', #17585 ) ;
#16127=ORIENTED_EDGE ( 'NONE', *, *, #702, .T. ) ;
#16165=AXIS2_PLACEMENT_3D ( 'NONE', #15848, #12512, #15942 ) ;
#16175=CARTESIAN_POINT ( 'NONE',  ( 1.500000000000000000, -4.769696007084728073, 15.00000000000000000 ) ) ;
#16210=DIRECTION ( 'NONE',  ( -0.000000000000000000, 1.000000000000000000, 0.000000000000000000 ) ) ;
#16287=ORIENTED_EDGE ( 'NONE', *, *, #16829, .T. ) ;
#16323=LINE ( 'NONE', #11349, #21283 ) ;
#16355=DIRECTION ( 'NONE',  ( -1.000000000000000000, 0.000000000000000000, 0.000000000000000000 ) ) ;
#16397=SHAPE_REPRESENTATION_RELATIONSHIP ( 'NONE' , 'NONE' ,  #14169, #2505 ) ;
#16432=ORIENTED_EDGE ( 'NONE', *, *, #15812, .T. ) ;
#16437=DIRECTION ( 'NONE',  ( 1.000000000000000000, 0.000000000000000000, 0.000000000000000000 ) ) ;
#16447=CARTESIAN_POINT ( 'NONE',  ( 2.799999999999996714, 60.00000000000000000, -15.00000000000000000 ) ) ;
#16619=AXIS2_PLACEMENT_3D ( 'NONE', #20893, #17694, #7757 ) ;
#16627=( GEOMETRIC_REPRESENTATION_CONTEXT ( 3 ) GLOBAL_UNCERTAINTY_ASSIGNED_CONTEXT ( ( #20067 ) ) GLOBAL_UNIT_ASSIGNED_CONTEXT ( ( #9761, #12861, #9319 ) ) REPRESENTATION_CONTEXT ( 'NONE', 'WORKASPACE' ) );
#16628=DIRECTION ( 'NONE',  ( 0.000000000000000000, 0.000000000000000000, -1.000000000000000000 ) ) ;
#16760=CARTESIAN_POINT ( 'NONE',  ( -5.000000000000000000, 5.000000000000000000, 9.999999999999998224 ) ) ;
#16770=DIRECTION ( 'NONE',  ( -0.000000000000000000, -0.000000000000000000, 1.000000000000000000 ) ) ;
#16772=AXIS2_PLACEMENT_3D ( 'NONE', #9224, #19506, #2715 ) ;
#16799=( NAMED_UNIT ( * ) SI_UNIT ( $, .STERADIAN. ) SOLID_ANGLE_UNIT ( ) );
#16829=EDGE_CURVE ( 'NONE', #21336, #8720, #9013, .T. ) ;
#16853=LINE ( 'NONE', #6597, #3208 ) ;
#16893=ADVANCED_FACE ( 'NONE', ( #20289 ), #3377, .T. ) ;
#16918=AXIS2_PLACEMENT_3D ( 'NONE', #5055, #16437, #8372 ) ;
#16978=ORIENTED_EDGE ( 'NONE', *, *, #11677, .T. ) ;
#16988=EDGE_CURVE ( 'NONE', #2130, #20275, #895, .T. ) ;
#17034=ORIENTED_EDGE ( 'NONE', *, *, #19100, .T. ) ;
#17080=EDGE_LOOP ( 'NONE', ( #19438, #15009, #12004, #2062, #16432, #7166 ) ) ;
#17085=DIRECTION ( 'NONE',  ( 1.000000000000000000, 0.000000000000000000, 0.000000000000000000 ) ) ;
#17145=ORIENTED_EDGE ( 'NONE', *, *, #11677, .F. ) ;
#17258=CARTESIAN_POINT ( 'NONE',  ( 0.000000000000000000, 60.00000000000000000, 9.999999999999998224 ) ) ;
#17279=CIRCLE ( 'NONE', #10203, 9.999999999999998224 ) ;
#17300=CIRCLE ( 'NONE', #11281, 9.999999999999998224 ) ;
#17316=ORIENTED_EDGE ( 'NONE', *, *, #16988, .F. ) ;
#17323=EDGE_CURVE ( 'NONE', #2849, #4329, #3401, .T. ) ;
#17359=ORIENTED_EDGE ( 'NONE', *, *, #8034, .F. ) ;
#17392=CARTESIAN_POINT ( 'NONE',  ( -1.500000000000000000, 0.000000000000000000, 5.000000000000000000 ) ) ;
#17497=DIRECTION ( 'NONE',  ( 1.000000000000000000, 0.000000000000000000, 0.000000000000000000 ) ) ;
#17522=PLANE ( 'NONE',  #15139 ) ;
#17537=AXIS2_PLACEMENT_3D ( 'NONE', #12926, #1337, #6541 ) ;
#17585=CARTESIAN_POINT ( 'NONE',  ( 1.500000000000000000, -7.000000000000000000, 5.000000000000000000 ) ) ;
#17609=LINE ( 'NONE', #14391, #15978 ) ;
#17625=LINE ( 'NONE', #21038, #19669 ) ;
#17635=DIRECTION ( 'NONE',  ( 1.000000000000000000, 0.000000000000000000, -0.000000000000000000 ) ) ;
#17648=CIRCLE ( 'NONE', #18000, 5.000000000000000000 ) ;
#17691=LINE ( 'NONE', #21118, #19691 ) ;
#17694=DIRECTION ( 'NONE',  ( -0.000000000000000000, -0.000000000000000000, 1.000000000000000000 ) ) ;
#17729=APPLICATION_CONTEXT ( 'automotive_design' ) ;
#17746=AXIS2_PLACEMENT_3D ( 'NONE', #6413, #16770, #18225 ) ;
#17769=DIRECTION ( 'NONE',  ( 0.000000000000000000, 1.000000000000000000, 0.000000000000000000 ) ) ;
#17817=EDGE_LOOP ( 'NONE', ( #19133, #1757, #2296, #2759, #13316, #9116 ) ) ;
#17887=CIRCLE ( 'NONE', #10109, 9.999999999999998224 ) ;
#17964=SURFACE_STYLE_USAGE ( .BOTH. , #1053 ) ;
#17981=ORIENTED_EDGE ( 'NONE', *, *, #1275, .T. ) ;
#18000=AXIS2_PLACEMENT_3D ( 'NONE', #13761, #21827, #20176 ) ;
#18045=DIRECTION ( 'NONE',  ( -0.000000000000000000, -0.000000000000000000, 1.000000000000000000 ) ) ;
#18138=PRODUCT ( 'planet connector', 'planet connector', '', ( #1791 ) ) ;
#18194=LINE ( 'NONE', #6484, #6049 ) ;
#18211=ORIENTED_EDGE ( 'NONE', *, *, #1999, .F. ) ;
#18225=DIRECTION ( 'NONE',  ( -1.000000000000000000, 0.000000000000000000, 0.000000000000000000 ) ) ;
#18251=SURFACE_SIDE_STYLE ('',( #13144 ) ) ;
#18278=DIRECTION ( 'NONE',  ( 0.000000000000000000, 0.000000000000000000, -1.000000000000000000 ) ) ;
#18287=LINE ( 'NONE', #1380, #14815 ) ;
#18321=ORIENTED_EDGE ( 'NONE', *, *, #908, .T. ) ;
#18340=LINE ( 'NONE', #6626, #8908 ) ;
#18362=AXIS2_PLACEMENT_3D ( 'NONE', #8215, #6694, #6578 ) ;
#18416=DIRECTION ( 'NONE',  ( 0.000000000000000000, -1.000000000000000000, 0.000000000000000000 ) ) ;
#18471=ORIENTED_EDGE ( 'NONE', *, *, #9433, .F. ) ;
#18485=AXIS2_PLACEMENT_3D ( 'NONE', #16760, #8368, #5053 ) ;
#18505=PLANE ( 'NONE',  #4743 ) ;
#18522=DIRECTION ( 'NONE',  ( 0.000000000000000000, 0.000000000000000000, 1.000000000000000000 ) ) ;
#18564=ORIENTED_EDGE ( 'NONE', *, *, #3234, .T. ) ;
#18623=CARTESIAN_POINT ( 'NONE',  ( 5.000000000000000000, 67.00000000000000000, 15.00000000000000000 ) ) ;
#18630=CIRCLE ( 'NONE', #21438, 5.000000000000000000 ) ;
#18649=VERTEX_POINT ( 'NONE', #7435 ) ;
#18687=( NAMED_UNIT ( * ) PLANE_ANGLE_UNIT ( ) SI_UNIT ( $, .RADIAN. ) );
#18707=CARTESIAN_POINT ( 'NONE',  ( 6.123233995736766282E-16, -5.000000000000000000, 3.000000000000002665 ) ) ;
#18727=EDGE_LOOP ( 'NONE', ( #2820, #15329 ) ) ;
#18748=ORIENTED_EDGE ( 'NONE', *, *, #5997, .T. ) ;
#18810=LINE ( 'NONE', #13833, #20102 ) ;
#18831=FACE_OUTER_BOUND ( 'NONE', #7537, .T. ) ;
#18881=CIRCLE ( 'NONE', #21003, 9.999999999999998224 ) ;
#18980=ORIENTED_EDGE ( 'NONE', *, *, #20997, .F. ) ;
#18985=VECTOR ( 'NONE', #1717, 1000.000000000000000 ) ;
#19050=CARTESIAN_POINT ( 'NONE',  ( 0.000000000000000000, 0.000000000000000000, 100.0000000000000000 ) ) ;
#19100=EDGE_CURVE ( 'NONE', #1080, #13824, #9834, .T. ) ;
#19130=CYLINDRICAL_SURFACE ( 'NONE', #16619, 2.799999999999996714 ) ;
#19133=ORIENTED_EDGE ( 'NONE', *, *, #19359, .F. ) ;
#19138=CARTESIAN_POINT ( 'NONE',  ( 2.000000000000000000, 67.00000000000000000, 15.00000000000000000 ) ) ;
#19161=VERTEX_POINT ( 'NONE', #14333 ) ;
#19304=ORIENTED_EDGE ( 'NONE', *, *, #21132, .T. ) ;
#19359=EDGE_CURVE ( 'NONE', #18649, #4329, #20509, .T. ) ;
#19370=AXIS2_PLACEMENT_3D ( 'NONE', #7710, #2618, #1074 ) ;
#19419=PLANE ( 'NONE',  #10046 ) ;
#19438=ORIENTED_EDGE ( 'NONE', *, *, #13563, .F. ) ;
#19463=CARTESIAN_POINT ( 'NONE',  ( -5.000000000000000000, 8.660254037844385522, 15.00000000000000000 ) ) ;
#19476=FACE_BOUND ( 'NONE', #4949, .T. ) ;
#19496=PRESENTATION_STYLE_ASSIGNMENT (( #17964 ) ) ;
#19506=DIRECTION ( 'NONE',  ( 0.000000000000000000, 0.000000000000000000, -1.000000000000000000 ) ) ;
#19520=EDGE_LOOP ( 'NONE', ( #21571, #18471, #237, #20209 ) ) ;
#19542=EDGE_CURVE ( 'NONE', #13591, #11791, #17279, .T. ) ;
#19558=CARTESIAN_POINT ( 'NONE',  ( -2.799999999999996714, 60.00000000000000000, -15.00000000000000000 ) ) ;
#19565=VECTOR ( 'NONE', #2197, 1000.000000000000000 ) ;
#19617=CYLINDRICAL_SURFACE ( 'NONE', #4860, 9.999999999999998224 ) ;
#19669=VECTOR ( 'NONE', #2810, 1000.000000000000000 ) ;
#19672=CARTESIAN_POINT ( 'NONE',  ( 2.000000000000000000, 70.00000000000000000, 9.999999999999998224 ) ) ;
#19679=DIRECTION ( 'NONE',  ( -1.000000000000000000, 0.000000000000000000, 0.000000000000000000 ) ) ;
#19691=VECTOR ( 'NONE', #5992, 1000.000000000000000 ) ;
#19720=VERTEX_POINT ( 'NONE', #11750 ) ;
#19853=VERTEX_POINT ( 'NONE', #13741 ) ;
#20010=CARTESIAN_POINT ( 'NONE',  ( -9.999999999999998224, 0.000000000000000000, 3.000000000000000000 ) ) ;
#20067=UNCERTAINTY_MEASURE_WITH_UNIT (LENGTH_MEASURE( 1.000000000000000082E-05 ), #9761, 'distance_accuracy_value', 'NONE');
#20102=VECTOR ( 'NONE', #7211, 1000.000000000000000 ) ;
#20162=EDGE_LOOP ( 'NONE', ( #8547, #9417, #4377, #10506 ) ) ;
#20176=DIRECTION ( 'NONE',  ( 1.000000000000000000, 0.000000000000000000, 0.000000000000000000 ) ) ;
#20187=DIRECTION ( 'NONE',  ( 0.000000000000000000, 0.000000000000000000, 1.000000000000000000 ) ) ;
#20209=ORIENTED_EDGE ( 'NONE', *, *, #19542, .T. ) ;
#20252=CARTESIAN_POINT ( 'NONE',  ( 1.500000000000000000, 0.000000000000000000, 15.00000000000000000 ) ) ;
#20275=VERTEX_POINT ( 'NONE', #15330 ) ;
#20289=FACE_OUTER_BOUND ( 'NONE', #13190, .T. ) ;
#20383=EDGE_CURVE ( 'NONE', #2563, #739, #12237, .T. ) ;
#20488=ORIENTED_EDGE ( 'NONE', *, *, #7549, .F. ) ;
#20489=DIRECTION ( 'NONE',  ( 0.000000000000000000, 0.000000000000000000, -1.000000000000000000 ) ) ;
#20491=EDGE_LOOP ( 'NONE', ( #12100, #1211, #13089, #7115, #7047 ) ) ;
#20509=LINE ( 'NONE', #503, #20792 ) ;
#20533=EDGE_CURVE ( 'NONE', #4414, #19161, #9455, .T. ) ;
#20552=DIRECTION ( 'NONE',  ( 1.000000000000000000, 0.000000000000000000, -0.000000000000000000 ) ) ;
#20553=PLANE ( 'NONE',  #8625 ) ;
#20554=DIRECTION ( 'NONE',  ( -0.000000000000000000, -0.000000000000000000, 1.000000000000000000 ) ) ;
#20610=FACE_BOUND ( 'NONE', #18727, .T. ) ;
#20630=DIRECTION ( 'NONE',  ( -1.000000000000000000, 0.000000000000000000, 0.000000000000000000 ) ) ;
#20650=DIRECTION ( 'NONE',  ( -1.000000000000000000, 0.000000000000000000, 0.000000000000000000 ) ) ;
#20659=CLOSED_SHELL ( 'NONE', ( #20954, #11542, #4037, #15525, #10273, #20805, #334, #12057, #5034, #10442, #14756, #13638, #8282, #12576, #7292, #3278, #8709, #5953, #16893 ) ) ;
#20685=DIRECTION ( 'NONE',  ( 1.000000000000000000, 0.000000000000000000, 0.000000000000000000 ) ) ;
#20766=DIRECTION ( 'NONE',  ( 0.000000000000000000, 0.000000000000000000, -1.000000000000000000 ) ) ;
#20792=VECTOR ( 'NONE', #5369, 1000.000000000000000 ) ;
#20805=ADVANCED_FACE ( 'NONE', ( #20610, #4025 ), #17522, .F. ) ;
#20867=DIRECTION ( 'NONE',  ( 0.000000000000000000, 0.000000000000000000, -1.000000000000000000 ) ) ;
#20870=DIRECTION ( 'NONE',  ( 0.000000000000000000, -1.000000000000000000, 0.000000000000000000 ) ) ;
#20893=CARTESIAN_POINT ( 'NONE',  ( 0.000000000000000000, 60.00000000000000000, -15.00000000000000000 ) ) ;
#20898=EDGE_CURVE ( 'NONE', #4038, #8443, #18287, .T. ) ;
#20899=DIRECTION ( 'NONE',  ( 1.000000000000000000, 0.000000000000000000, 0.000000000000000000 ) ) ;
#20954=ADVANCED_FACE ( 'NONE', ( #11971 ), #1473, .T. ) ;
#20956=FACE_OUTER_BOUND ( 'NONE', #19520, .T. ) ;
#20997=EDGE_CURVE ( 'NONE', #14473, #8443, #17300, .T. ) ;
#21003=AXIS2_PLACEMENT_3D ( 'NONE', #21414, #4624, #11581 ) ;
#21038=CARTESIAN_POINT ( 'NONE',  ( 2.799999999999996714, 60.00000000000000000, -15.00000000000000000 ) ) ;
#21084=FACE_OUTER_BOUND ( 'NONE', #11134, .T. ) ;
#21118=CARTESIAN_POINT ( 'NONE',  ( 2.000000000000000000, 70.00000000000000000, 9.999999999999998224 ) ) ;
#21122=FACE_OUTER_BOUND ( 'NONE', #15125, .T. ) ;
#21132=EDGE_CURVE ( 'NONE', #1388, #2507, #6028, .T. ) ;
#21150=DIRECTION ( 'NONE',  ( 1.000000000000000000, 0.000000000000000000, -0.000000000000000000 ) ) ;
#21165=ORIENTED_EDGE ( 'NONE', *, *, #8007, .T. ) ;
#21170=DIRECTION ( 'NONE',  ( -1.000000000000000000, 0.000000000000000000, 0.000000000000000000 ) ) ;
#21194=ORIENTED_EDGE ( 'NONE', *, *, #4288, .F. ) ;
#21283=VECTOR ( 'NONE', #15896, 1000.000000000000000 ) ;
#21311=ORIENTED_EDGE ( 'NONE', *, *, #9433, .T. ) ;
#21315=ORIENTED_EDGE ( 'NONE', *, *, #3634, .T. ) ;
#21336=VERTEX_POINT ( 'NONE', #19463 ) ;
#21352=ORIENTED_EDGE ( 'NONE', *, *, #702, .F. ) ;
#21365=EDGE_CURVE ( 'NONE', #19161, #14453, #3894, .T. ) ;
#21377=AXIS2_PLACEMENT_3D ( 'NONE', #4551, #1017, #19679 ) ;
#21414=CARTESIAN_POINT ( 'NONE',  ( 0.000000000000000000, 0.000000000000000000, 15.00000000000000000 ) ) ;
#21438=AXIS2_PLACEMENT_3D ( 'NONE', #1010, #12386, #779 ) ;
#21546=EDGE_LOOP ( 'NONE', ( #11329, #7027, #9118, #13575, #260, #2133 ) ) ;
#21571=ORIENTED_EDGE ( 'NONE', *, *, #1275, .F. ) ;
#21706=AXIS2_PLACEMENT_3D ( 'NONE', #4456, #3014, #21150 ) ;
#21804=DIRECTION ( 'NONE',  ( 0.000000000000000000, 0.000000000000000000, 1.000000000000000000 ) ) ;
#21809=CIRCLE ( 'NONE', #16165, 9.999999999999998224 ) ;
#21827=DIRECTION ( 'NONE',  ( 0.000000000000000000, 0.000000000000000000, 1.000000000000000000 ) ) ;
#21837=CARTESIAN_POINT ( 'NONE',  ( 0.000000000000000000, 0.000000000000000000, 0.000000000000000000 ) ) ;
#21855=LINE ( 'NONE', #6954, #9967 ) ;
ENDSEC;
END-ISO-10303-21;
